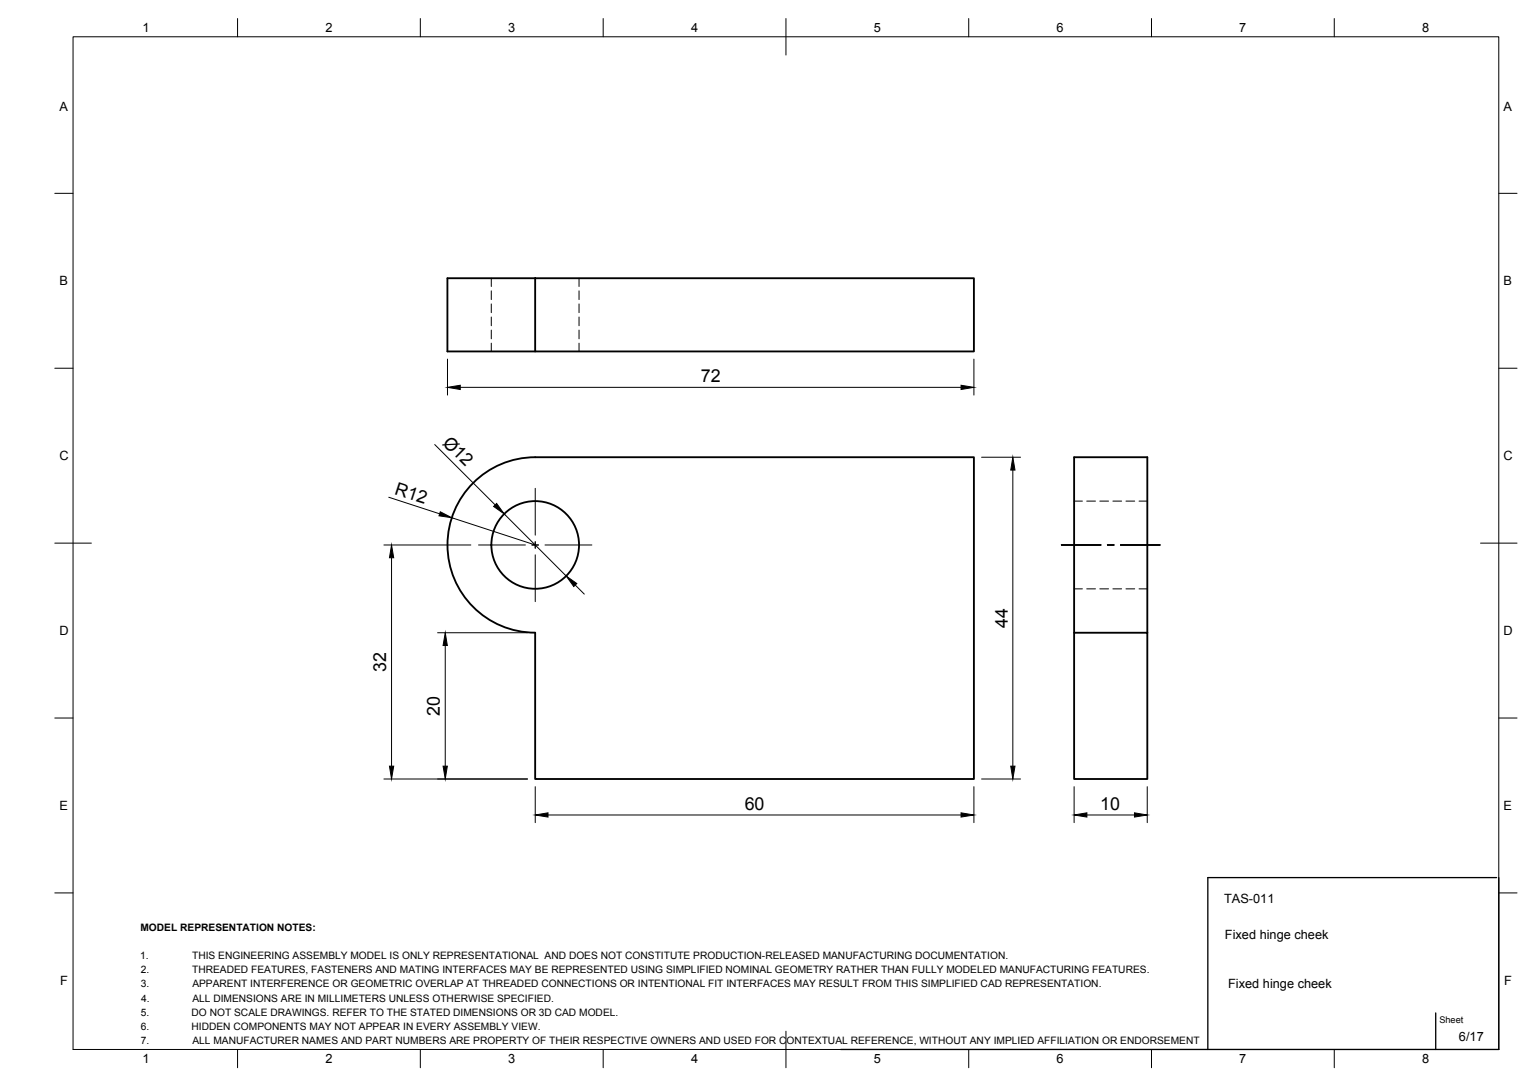
ISO-10303-21;
HEADER;
/* Generated by software containing ST-Developer
 * from STEP Tools, Inc. (www.steptools.com) 
 */

FILE_DESCRIPTION(
/* description */ (
'Independent manual bench leaf bending machine,200mm work width. Fabri
cated welded frame and folding leaf, repeated bushed and fully retaine
d hinge hardware, two handles with bonded grips, beveled clamping beam
 and modeledM12 clamp screws.2mm omitted-workpiece assembly reference 
gap, not a capacity claim. Native135deg hinge travel. Weld sizing, pro
duction fits, material condition, bending capacity, strength and life 
unassigned.'),
/* implementation_level */ '2;1');

FILE_NAME(
/* name */ 'Fixed hinge cheek.step',
/* time_stamp */ '2026-11-14T09:11:34-08:00',
/* author */ (''),
/* organization */ (''),
/* preprocessor_version */ 'ST-DEVELOPER v20.2',
/* originating_system */ 'Autodesk Translation Framework v15.17.0.0',
/* authorisation */ '');

FILE_SCHEMA (('AUTOMOTIVE_DESIGN { 1 0 10303 214 3 1 1 }'));
ENDSEC;

DATA;
#10=MECHANICAL_DESIGN_GEOMETRIC_PRESENTATION_REPRESENTATION('',(#451),#37701);
#415=SHAPE_REPRESENTATION_RELATIONSHIP('SRR','None',#37784,#433);
#433=ADVANCED_BREP_SHAPE_REPRESENTATION('',(#469),#37688);
#451=STYLED_ITEM('',(#37878),#469);
#469=MANIFOLD_SOLID_BREP('Body1',#4149);
#498=FACE_BOUND('',#883,.T.);
#499=FACE_BOUND('',#885,.T.);
#546=PLANE('',#4445);
#547=PLANE('',#4446);
#548=PLANE('',#4447);
#549=PLANE('',#4448);
#550=PLANE('',#4452);
#551=PLANE('',#4453);
#648=FACE_OUTER_BOUND('',#876,.T.);
#649=FACE_OUTER_BOUND('',#877,.T.);
#650=FACE_OUTER_BOUND('',#878,.T.);
#651=FACE_OUTER_BOUND('',#879,.T.);
#652=FACE_OUTER_BOUND('',#880,.T.);
#653=FACE_OUTER_BOUND('',#881,.T.);
#654=FACE_OUTER_BOUND('',#882,.T.);
#655=FACE_OUTER_BOUND('',#884,.T.);
#876=EDGE_LOOP('',(#2847,#2848,#2849,#2850));
#877=EDGE_LOOP('',(#2851,#2852,#2853,#2854));
#878=EDGE_LOOP('',(#2855,#2856,#2857,#2858));
#879=EDGE_LOOP('',(#2859,#2860,#2861,#2862));
#880=EDGE_LOOP('',(#2863,#2864,#2865,#2866));
#881=EDGE_LOOP('',(#2867,#2868,#2869,#2870));
#882=EDGE_LOOP('',(#2871,#2872,#2873,#2874,#2875));
#883=EDGE_LOOP('',(#2876));
#884=EDGE_LOOP('',(#2877,#2878,#2879,#2880,#2881));
#885=EDGE_LOOP('',(#2882));
#1136=LINE('',#5877,#1385);
#1137=LINE('',#5882,#1386);
#1138=LINE('',#5884,#1387);
#1139=LINE('',#5886,#1388);
#1140=LINE('',#5887,#1389);
#1141=LINE('',#5890,#1390);
#1142=LINE('',#5892,#1391);
#1143=LINE('',#5893,#1392);
#1144=LINE('',#5896,#1393);
#1145=LINE('',#5898,#1394);
#1146=LINE('',#5899,#1395);
#1147=LINE('',#5902,#1396);
#1148=LINE('',#5904,#1397);
#1149=LINE('',#5905,#1398);
#1385=VECTOR('',#4949,6.);
#1386=VECTOR('',#4954,10.);
#1387=VECTOR('',#4955,10.);
#1388=VECTOR('',#4956,10.);
#1389=VECTOR('',#4957,10.);
#1390=VECTOR('',#4960,10.);
#1391=VECTOR('',#4961,10.);
#1392=VECTOR('',#4962,10.);
#1393=VECTOR('',#4965,10.);
#1394=VECTOR('',#4966,10.);
#1395=VECTOR('',#4967,10.);
#1396=VECTOR('',#4970,10.);
#1397=VECTOR('',#4971,10.);
#1398=VECTOR('',#4972,10.);
#1582=CIRCLE('',#4443,6.);
#1583=CIRCLE('',#4444,6.);
#1584=CIRCLE('',#4450,12.);
#1585=CIRCLE('',#4451,12.);
#1705=VERTEX_POINT('',#5874);
#1706=VERTEX_POINT('',#5876);
#1707=VERTEX_POINT('',#5880);
#1708=VERTEX_POINT('',#5881);
#1709=VERTEX_POINT('',#5883);
#1710=VERTEX_POINT('',#5885);
#1711=VERTEX_POINT('',#5889);
#1712=VERTEX_POINT('',#5891);
#1713=VERTEX_POINT('',#5895);
#1714=VERTEX_POINT('',#5897);
#1715=VERTEX_POINT('',#5901);
#1716=VERTEX_POINT('',#5903);
#2157=EDGE_CURVE('',#1705,#1705,#1582,.T.);
#2158=EDGE_CURVE('',#1705,#1706,#1136,.T.);
#2159=EDGE_CURVE('',#1706,#1706,#1583,.T.);
#2160=EDGE_CURVE('',#1707,#1708,#1137,.T.);
#2161=EDGE_CURVE('',#1707,#1709,#1138,.T.);
#2162=EDGE_CURVE('',#1710,#1709,#1139,.T.);
#2163=EDGE_CURVE('',#1708,#1710,#1140,.T.);
#2164=EDGE_CURVE('',#1708,#1711,#1141,.T.);
#2165=EDGE_CURVE('',#1712,#1710,#1142,.T.);
#2166=EDGE_CURVE('',#1711,#1712,#1143,.T.);
#2167=EDGE_CURVE('',#1711,#1713,#1144,.T.);
#2168=EDGE_CURVE('',#1714,#1712,#1145,.T.);
#2169=EDGE_CURVE('',#1713,#1714,#1146,.T.);
#2170=EDGE_CURVE('',#1713,#1715,#1147,.T.);
#2171=EDGE_CURVE('',#1716,#1714,#1148,.T.);
#2172=EDGE_CURVE('',#1715,#1716,#1149,.T.);
#2173=EDGE_CURVE('',#1707,#1715,#1584,.T.);
#2174=EDGE_CURVE('',#1709,#1716,#1585,.T.);
#2847=ORIENTED_EDGE('',*,*,#2157,.F.);
#2848=ORIENTED_EDGE('',*,*,#2158,.T.);
#2849=ORIENTED_EDGE('',*,*,#2159,.F.);
#2850=ORIENTED_EDGE('',*,*,#2158,.F.);
#2851=ORIENTED_EDGE('',*,*,#2160,.F.);
#2852=ORIENTED_EDGE('',*,*,#2161,.T.);
#2853=ORIENTED_EDGE('',*,*,#2162,.F.);
#2854=ORIENTED_EDGE('',*,*,#2163,.F.);
#2855=ORIENTED_EDGE('',*,*,#2164,.F.);
#2856=ORIENTED_EDGE('',*,*,#2163,.T.);
#2857=ORIENTED_EDGE('',*,*,#2165,.F.);
#2858=ORIENTED_EDGE('',*,*,#2166,.F.);
#2859=ORIENTED_EDGE('',*,*,#2167,.F.);
#2860=ORIENTED_EDGE('',*,*,#2166,.T.);
#2861=ORIENTED_EDGE('',*,*,#2168,.F.);
#2862=ORIENTED_EDGE('',*,*,#2169,.F.);
#2863=ORIENTED_EDGE('',*,*,#2170,.F.);
#2864=ORIENTED_EDGE('',*,*,#2169,.T.);
#2865=ORIENTED_EDGE('',*,*,#2171,.F.);
#2866=ORIENTED_EDGE('',*,*,#2172,.F.);
#2867=ORIENTED_EDGE('',*,*,#2173,.T.);
#2868=ORIENTED_EDGE('',*,*,#2172,.T.);
#2869=ORIENTED_EDGE('',*,*,#2174,.F.);
#2870=ORIENTED_EDGE('',*,*,#2161,.F.);
#2871=ORIENTED_EDGE('',*,*,#2174,.T.);
#2872=ORIENTED_EDGE('',*,*,#2171,.T.);
#2873=ORIENTED_EDGE('',*,*,#2168,.T.);
#2874=ORIENTED_EDGE('',*,*,#2165,.T.);
#2875=ORIENTED_EDGE('',*,*,#2162,.T.);
#2876=ORIENTED_EDGE('',*,*,#2157,.T.);
#2877=ORIENTED_EDGE('',*,*,#2173,.F.);
#2878=ORIENTED_EDGE('',*,*,#2160,.T.);
#2879=ORIENTED_EDGE('',*,*,#2164,.T.);
#2880=ORIENTED_EDGE('',*,*,#2167,.T.);
#2881=ORIENTED_EDGE('',*,*,#2170,.T.);
#2882=ORIENTED_EDGE('',*,*,#2159,.T.);
#3827=CYLINDRICAL_SURFACE('',#4442,6.);
#3828=CYLINDRICAL_SURFACE('',#4449,12.);
#3978=ADVANCED_FACE('',(#648),#3827,.F.);
#3979=ADVANCED_FACE('',(#649),#546,.T.);
#3980=ADVANCED_FACE('',(#650),#547,.T.);
#3981=ADVANCED_FACE('',(#651),#548,.T.);
#3982=ADVANCED_FACE('',(#652),#549,.T.);
#3983=ADVANCED_FACE('',(#653),#3828,.T.);
#3984=ADVANCED_FACE('',(#654,#498),#550,.T.);
#3985=ADVANCED_FACE('',(#655,#499),#551,.F.);
#4149=CLOSED_SHELL('',(#3978,#3979,#3980,#3981,#3982,#3983,#3984,#3985));
#4441=AXIS2_PLACEMENT_3D('',#5872,#4943,#4944);
#4442=AXIS2_PLACEMENT_3D('',#5873,#4945,#4946);
#4443=AXIS2_PLACEMENT_3D('',#5875,#4947,#4948);
#4444=AXIS2_PLACEMENT_3D('',#5878,#4950,#4951);
#4445=AXIS2_PLACEMENT_3D('',#5879,#4952,#4953);
#4446=AXIS2_PLACEMENT_3D('',#5888,#4958,#4959);
#4447=AXIS2_PLACEMENT_3D('',#5894,#4963,#4964);
#4448=AXIS2_PLACEMENT_3D('',#5900,#4968,#4969);
#4449=AXIS2_PLACEMENT_3D('',#5906,#4973,#4974);
#4450=AXIS2_PLACEMENT_3D('',#5907,#4975,#4976);
#4451=AXIS2_PLACEMENT_3D('',#5908,#4977,#4978);
#4452=AXIS2_PLACEMENT_3D('',#5909,#4979,#4980);
#4453=AXIS2_PLACEMENT_3D('',#5910,#4981,#4982);
#4943=DIRECTION('axis',(0.,0.,1.));
#4944=DIRECTION('refdir',(1.,0.,0.));
#4945=DIRECTION('center_axis',(0.,-1.,0.));
#4946=DIRECTION('ref_axis',(0.,0.,1.));
#4947=DIRECTION('center_axis',(0.,-1.,0.));
#4948=DIRECTION('ref_axis',(0.,0.,1.));
#4949=DIRECTION('',(0.,-1.,0.));
#4950=DIRECTION('center_axis',(0.,1.,0.));
#4951=DIRECTION('ref_axis',(0.,0.,1.));
#4952=DIRECTION('center_axis',(0.,0.,1.));
#4953=DIRECTION('ref_axis',(1.,0.,0.));
#4954=DIRECTION('',(-1.,0.,0.));
#4955=DIRECTION('',(0.,1.,0.));
#4956=DIRECTION('',(1.,0.,0.));
#4957=DIRECTION('',(0.,1.,0.));
#4958=DIRECTION('center_axis',(-1.,0.,0.));
#4959=DIRECTION('ref_axis',(0.,0.,1.));
#4960=DIRECTION('',(0.,0.,-1.));
#4961=DIRECTION('',(0.,0.,1.));
#4962=DIRECTION('',(0.,1.,0.));
#4963=DIRECTION('center_axis',(0.,0.,-1.));
#4964=DIRECTION('ref_axis',(-1.,0.,0.));
#4965=DIRECTION('',(1.,0.,0.));
#4966=DIRECTION('',(-1.,0.,0.));
#4967=DIRECTION('',(0.,1.,0.));
#4968=DIRECTION('center_axis',(1.,0.,0.));
#4969=DIRECTION('ref_axis',(0.,0.,-1.));
#4970=DIRECTION('',(0.,0.,1.));
#4971=DIRECTION('',(0.,0.,-1.));
#4972=DIRECTION('',(0.,1.,0.));
#4973=DIRECTION('center_axis',(0.,1.,0.));
#4974=DIRECTION('ref_axis',(3.70074341541719E-16,0.,1.));
#4975=DIRECTION('center_axis',(0.,1.,0.));
#4976=DIRECTION('ref_axis',(3.70074341541719E-16,0.,1.));
#4977=DIRECTION('center_axis',(0.,1.,0.));
#4978=DIRECTION('ref_axis',(3.70074341541719E-16,0.,1.));
#4979=DIRECTION('center_axis',(0.,1.,0.));
#4980=DIRECTION('ref_axis',(1.,0.,0.));
#4981=DIRECTION('center_axis',(0.,1.,0.));
#4982=DIRECTION('ref_axis',(1.,0.,0.));
#5872=CARTESIAN_POINT('',(0.,0.,0.));
#5873=CARTESIAN_POINT('Origin',(0.,5.,42.));
#5874=CARTESIAN_POINT('',(7.34788079488412E-16,10.,36.));
#5875=CARTESIAN_POINT('Origin',(0.,10.,42.));
#5876=CARTESIAN_POINT('',(7.34788079488412E-16,0.,36.));
#5877=CARTESIAN_POINT('',(7.34788079488412E-16,5.,36.));
#5878=CARTESIAN_POINT('Origin',(0.,0.,42.));
#5879=CARTESIAN_POINT('Origin',(-60.,0.,54.));
#5880=CARTESIAN_POINT('',(0.,0.,54.));
#5881=CARTESIAN_POINT('',(-60.,0.,54.));
#5882=CARTESIAN_POINT('',(0.,0.,54.));
#5883=CARTESIAN_POINT('',(0.,10.,54.));
#5884=CARTESIAN_POINT('',(0.,0.,54.));
#5885=CARTESIAN_POINT('',(-60.,10.,54.));
#5886=CARTESIAN_POINT('',(0.,10.,54.));
#5887=CARTESIAN_POINT('',(-60.,0.,54.));
#5888=CARTESIAN_POINT('Origin',(-60.,0.,10.));
#5889=CARTESIAN_POINT('',(-60.,0.,10.));
#5890=CARTESIAN_POINT('',(-60.,0.,54.));
#5891=CARTESIAN_POINT('',(-60.,10.,10.));
#5892=CARTESIAN_POINT('',(-60.,10.,54.));
#5893=CARTESIAN_POINT('',(-60.,0.,10.));
#5894=CARTESIAN_POINT('Origin',(0.,0.,10.));
#5895=CARTESIAN_POINT('',(0.,0.,10.));
#5896=CARTESIAN_POINT('',(-60.,0.,10.));
#5897=CARTESIAN_POINT('',(0.,10.,10.));
#5898=CARTESIAN_POINT('',(-60.,10.,10.));
#5899=CARTESIAN_POINT('',(0.,0.,10.));
#5900=CARTESIAN_POINT('Origin',(0.,0.,30.));
#5901=CARTESIAN_POINT('',(-7.41220803802443E-15,0.,30.));
#5902=CARTESIAN_POINT('',(0.,0.,10.));
#5903=CARTESIAN_POINT('',(-7.41220803802443E-15,10.,30.));
#5904=CARTESIAN_POINT('',(0.,10.,10.));
#5905=CARTESIAN_POINT('',(-7.41220803802443E-15,0.,30.));
#5906=CARTESIAN_POINT('Origin',(-4.44089209850063E-15,0.,42.));
#5907=CARTESIAN_POINT('Origin',(-4.44089209850063E-15,0.,42.));
#5908=CARTESIAN_POINT('Origin',(-4.44089209850063E-15,10.,42.));
#5909=CARTESIAN_POINT('Origin',(-24.,10.,32.));
#5910=CARTESIAN_POINT('Origin',(-24.,0.,32.));
#37668=UNCERTAINTY_MEASURE_WITH_UNIT(LENGTH_MEASURE(0.01),#37702,
'DISTANCE_ACCURACY_VALUE',
'Maximum model space distance between geometric entities at asserted c
onnectivities');
#37681=UNCERTAINTY_MEASURE_WITH_UNIT(LENGTH_MEASURE(0.01),#37702,
'DISTANCE_ACCURACY_VALUE',
'Maximum model space distance between geometric entities at asserted c
onnectivities');
#37688=(
GEOMETRIC_REPRESENTATION_CONTEXT(3)
GLOBAL_UNCERTAINTY_ASSIGNED_CONTEXT((#37668))
GLOBAL_UNIT_ASSIGNED_CONTEXT((#37702,#37704,#37705))
REPRESENTATION_CONTEXT('','3D')
);
#37701=(
GEOMETRIC_REPRESENTATION_CONTEXT(3)
GLOBAL_UNCERTAINTY_ASSIGNED_CONTEXT((#37681))
GLOBAL_UNIT_ASSIGNED_CONTEXT((#37702,#37704,#37705))
REPRESENTATION_CONTEXT('','3D')
);
#37702=(
LENGTH_UNIT()
NAMED_UNIT(*)
SI_UNIT(.MILLI.,.METRE.)
);
#37704=(
NAMED_UNIT(*)
PLANE_ANGLE_UNIT()
SI_UNIT($,.RADIAN.)
);
#37705=(
NAMED_UNIT(*)
SI_UNIT($,.STERADIAN.)
SOLID_ANGLE_UNIT()
);
#37712=SHAPE_DEFINITION_REPRESENTATION(#37731,#37784);
#37731=PRODUCT_DEFINITION_SHAPE('',$,#37804);
#37784=SHAPE_REPRESENTATION('',(#4441),#37688);
#37797=PRODUCT_DEFINITION_CONTEXT('part definition',#37856,'design');
#37804=PRODUCT_DEFINITION('Fixed hinge cheek','Fixed hinge cheek',#37823,
#37797);
#37823=PRODUCT_DEFINITION_FORMATION('',$,#37864);
#37856=APPLICATION_CONTEXT(
'Core Data for Automotive Mechanical Design Process');
#37857=PRODUCT_CONTEXT('part definition',#37856,'mechanical');
#37864=PRODUCT('Fixed hinge cheek','Fixed hinge cheek',$,(#37857));
#37878=PRESENTATION_STYLE_ASSIGNMENT((#37886));
#37886=SURFACE_STYLE_USAGE(.BOTH.,#37894);
#37894=SURFACE_SIDE_STYLE('',(#37902));
#37902=SURFACE_STYLE_FILL_AREA(#37910);
#37910=FILL_AREA_STYLE('Opaque(23,69,131)',(#37918));
#37918=FILL_AREA_STYLE_COLOUR('Opaque(23,69,131)',#37926);
#37926=COLOUR_RGB('Opaque(23,69,131)',0.0901960784313725,0.270588235294118,
0.513725490196078);
ENDSEC;
END-ISO-10303-21;
